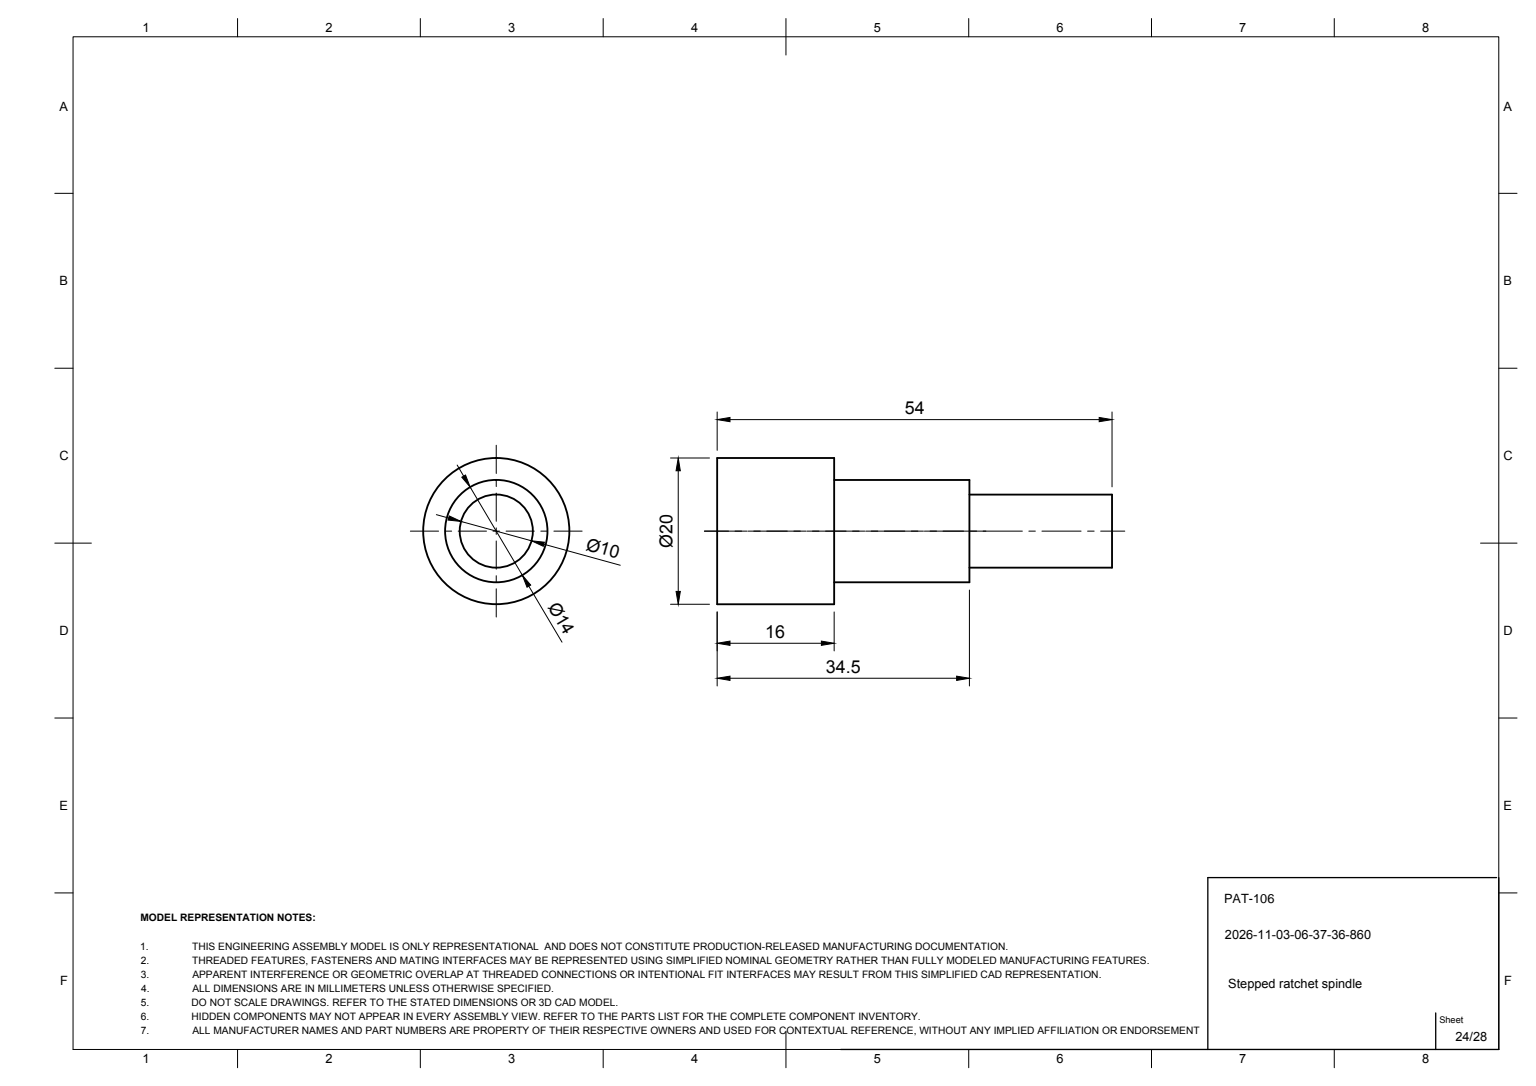
ISO-10303-21;
HEADER;
/* Generated by software containing ST-Developer
 * from STEP Tools, Inc. (www.steptools.com) 
 */

FILE_DESCRIPTION(
/* description */ ('Torsion-spring ratchet demonstrator'),
/* implementation_level */ '2;1');

FILE_NAME(
/* name */ 'Stepped ratchet spindle.step',
/* time_stamp */ '2026-10-29T17:29:17-07:00',
/* author */ (''),
/* organization */ (''),
/* preprocessor_version */ 'ST-DEVELOPER v20.2',
/* originating_system */ 'Autodesk Translation Framework v15.17.0.0',
/* authorisation */ '');

FILE_SCHEMA (('AUTOMOTIVE_DESIGN { 1 0 10303 214 3 1 1 }'));
ENDSEC;

DATA;
#10=MECHANICAL_DESIGN_GEOMETRIC_PRESENTATION_REPRESENTATION('',(#308),#11258);
#252=SHAPE_REPRESENTATION_RELATIONSHIP('SRR','None',#11380,#276);
#276=ADVANCED_BREP_SHAPE_REPRESENTATION('',(#338),#11250);
#308=STYLED_ITEM('',(#11577),#338);
#338=MANIFOLD_SOLID_BREP('Body1',#5181);
#420=FACE_BOUND('',#1196,.T.);
#421=FACE_BOUND('',#1199,.T.);
#530=PLANE('',#5896);
#531=PLANE('',#5901);
#532=PLANE('',#5907);
#533=PLANE('',#5908);
#815=FACE_OUTER_BOUND('',#1195,.T.);
#816=FACE_OUTER_BOUND('',#1197,.T.);
#817=FACE_OUTER_BOUND('',#1198,.T.);
#818=FACE_OUTER_BOUND('',#1200,.T.);
#819=FACE_OUTER_BOUND('',#1201,.T.);
#820=FACE_OUTER_BOUND('',#1202,.T.);
#821=FACE_OUTER_BOUND('',#1203,.T.);
#1195=EDGE_LOOP('',(#4212));
#1196=EDGE_LOOP('',(#4213));
#1197=EDGE_LOOP('',(#4214,#4215,#4216,#4217));
#1198=EDGE_LOOP('',(#4218));
#1199=EDGE_LOOP('',(#4219));
#1200=EDGE_LOOP('',(#4220,#4221,#4222,#4223));
#1201=EDGE_LOOP('',(#4224,#4225,#4226,#4227));
#1202=EDGE_LOOP('',(#4228));
#1203=EDGE_LOOP('',(#4229));
#1481=LINE('',#10498,#1864);
#1482=LINE('',#10505,#1865);
#1483=LINE('',#10508,#1866);
#1864=VECTOR('',#7118,1.);
#1865=VECTOR('',#7127,0.7);
#1866=VECTOR('',#7130,0.5);
#2295=CIRCLE('',#5897,1.);
#2296=CIRCLE('',#5898,0.7);
#2297=CIRCLE('',#5900,1.);
#2298=CIRCLE('',#5902,0.7);
#2299=CIRCLE('',#5903,0.5);
#2300=CIRCLE('',#5906,0.5);
#2599=VERTEX_POINT('',#10491);
#2600=VERTEX_POINT('',#10493);
#2601=VERTEX_POINT('',#10496);
#2602=VERTEX_POINT('',#10500);
#2603=VERTEX_POINT('',#10502);
#2604=VERTEX_POINT('',#10507);
#3166=EDGE_CURVE('',#2599,#2599,#2295,.T.);
#3167=EDGE_CURVE('',#2600,#2600,#2296,.T.);
#3168=EDGE_CURVE('',#2601,#2601,#2297,.T.);
#3169=EDGE_CURVE('',#2601,#2599,#1481,.T.);
#3170=EDGE_CURVE('',#2602,#2602,#2298,.T.);
#3171=EDGE_CURVE('',#2603,#2603,#2299,.T.);
#3172=EDGE_CURVE('',#2600,#2602,#1482,.T.);
#3173=EDGE_CURVE('',#2603,#2604,#1483,.T.);
#3174=EDGE_CURVE('',#2604,#2604,#2300,.T.);
#4212=ORIENTED_EDGE('',*,*,#3166,.F.);
#4213=ORIENTED_EDGE('',*,*,#3167,.T.);
#4214=ORIENTED_EDGE('',*,*,#3168,.F.);
#4215=ORIENTED_EDGE('',*,*,#3169,.T.);
#4216=ORIENTED_EDGE('',*,*,#3166,.T.);
#4217=ORIENTED_EDGE('',*,*,#3169,.F.);
#4218=ORIENTED_EDGE('',*,*,#3170,.F.);
#4219=ORIENTED_EDGE('',*,*,#3171,.F.);
#4220=ORIENTED_EDGE('',*,*,#3167,.F.);
#4221=ORIENTED_EDGE('',*,*,#3172,.T.);
#4222=ORIENTED_EDGE('',*,*,#3170,.T.);
#4223=ORIENTED_EDGE('',*,*,#3172,.F.);
#4224=ORIENTED_EDGE('',*,*,#3171,.T.);
#4225=ORIENTED_EDGE('',*,*,#3173,.T.);
#4226=ORIENTED_EDGE('',*,*,#3174,.T.);
#4227=ORIENTED_EDGE('',*,*,#3173,.F.);
#4228=ORIENTED_EDGE('',*,*,#3168,.T.);
#4229=ORIENTED_EDGE('',*,*,#3174,.F.);
#4832=CYLINDRICAL_SURFACE('',#5899,1.);
#4833=CYLINDRICAL_SURFACE('',#5904,0.7);
#4834=CYLINDRICAL_SURFACE('',#5905,0.5);
#5041=ADVANCED_FACE('',(#815,#420),#530,.F.);
#5042=ADVANCED_FACE('',(#816),#4832,.T.);
#5043=ADVANCED_FACE('',(#817,#421),#531,.F.);
#5044=ADVANCED_FACE('',(#818),#4833,.T.);
#5045=ADVANCED_FACE('',(#819),#4834,.T.);
#5046=ADVANCED_FACE('',(#820),#532,.T.);
#5047=ADVANCED_FACE('',(#821),#533,.F.);
#5181=CLOSED_SHELL('',(#5041,#5042,#5043,#5044,#5045,#5046,#5047));
#5895=AXIS2_PLACEMENT_3D('',#10489,#7106,#7107);
#5896=AXIS2_PLACEMENT_3D('',#10490,#7108,#7109);
#5897=AXIS2_PLACEMENT_3D('',#10492,#7110,#7111);
#5898=AXIS2_PLACEMENT_3D('',#10494,#7112,#7113);
#5899=AXIS2_PLACEMENT_3D('',#10495,#7114,#7115);
#5900=AXIS2_PLACEMENT_3D('',#10497,#7116,#7117);
#5901=AXIS2_PLACEMENT_3D('',#10499,#7119,#7120);
#5902=AXIS2_PLACEMENT_3D('',#10501,#7121,#7122);
#5903=AXIS2_PLACEMENT_3D('',#10503,#7123,#7124);
#5904=AXIS2_PLACEMENT_3D('',#10504,#7125,#7126);
#5905=AXIS2_PLACEMENT_3D('',#10506,#7128,#7129);
#5906=AXIS2_PLACEMENT_3D('',#10509,#7131,#7132);
#5907=AXIS2_PLACEMENT_3D('',#10510,#7133,#7134);
#5908=AXIS2_PLACEMENT_3D('',#10511,#7135,#7136);
#7106=DIRECTION('axis',(0.,0.,1.));
#7107=DIRECTION('refdir',(1.,0.,0.));
#7108=DIRECTION('center_axis',(0.,0.,1.));
#7109=DIRECTION('ref_axis',(1.,0.,0.));
#7110=DIRECTION('center_axis',(0.,0.,1.));
#7111=DIRECTION('ref_axis',(1.,0.,0.));
#7112=DIRECTION('center_axis',(0.,0.,1.));
#7113=DIRECTION('ref_axis',(1.,0.,0.));
#7114=DIRECTION('center_axis',(0.,0.,1.));
#7115=DIRECTION('ref_axis',(1.,0.,0.));
#7116=DIRECTION('center_axis',(0.,0.,1.));
#7117=DIRECTION('ref_axis',(1.,0.,0.));
#7118=DIRECTION('',(0.,0.,-1.));
#7119=DIRECTION('center_axis',(0.,0.,1.));
#7120=DIRECTION('ref_axis',(1.,0.,0.));
#7121=DIRECTION('center_axis',(0.,0.,1.));
#7122=DIRECTION('ref_axis',(1.,0.,0.));
#7123=DIRECTION('center_axis',(0.,0.,-1.));
#7124=DIRECTION('ref_axis',(1.,0.,0.));
#7125=DIRECTION('center_axis',(0.,0.,1.));
#7126=DIRECTION('ref_axis',(1.,0.,0.));
#7127=DIRECTION('',(0.,0.,-1.));
#7128=DIRECTION('center_axis',(0.,0.,1.));
#7129=DIRECTION('ref_axis',(1.,0.,0.));
#7130=DIRECTION('',(0.,0.,-1.));
#7131=DIRECTION('center_axis',(0.,0.,1.));
#7132=DIRECTION('ref_axis',(1.,0.,0.));
#7133=DIRECTION('center_axis',(0.,0.,1.));
#7134=DIRECTION('ref_axis',(1.,0.,0.));
#7135=DIRECTION('center_axis',(0.,0.,1.));
#7136=DIRECTION('ref_axis',(1.,0.,0.));
#10489=CARTESIAN_POINT('',(0.,0.,0.));
#10490=CARTESIAN_POINT('Origin',(0.,0.,4.8));
#10491=CARTESIAN_POINT('',(-1.,-1.22464679914735E-16,4.8));
#10492=CARTESIAN_POINT('Origin',(0.,0.,4.8));
#10493=CARTESIAN_POINT('',(-0.7,-8.57252759403147E-17,4.8));
#10494=CARTESIAN_POINT('Origin',(0.,0.,4.8));
#10495=CARTESIAN_POINT('Origin',(0.,0.,4.8));
#10496=CARTESIAN_POINT('',(-1.,-1.22464679914735E-16,6.4));
#10497=CARTESIAN_POINT('Origin',(0.,0.,6.4));
#10498=CARTESIAN_POINT('',(-1.,-1.22464679914735E-16,4.8));
#10499=CARTESIAN_POINT('Origin',(0.,0.,2.95));
#10500=CARTESIAN_POINT('',(-0.7,-8.57252759403147E-17,2.95));
#10501=CARTESIAN_POINT('Origin',(0.,0.,2.95));
#10502=CARTESIAN_POINT('',(-0.5,6.12323399573677E-17,2.95));
#10503=CARTESIAN_POINT('Origin',(0.,0.,2.95));
#10504=CARTESIAN_POINT('Origin',(0.,0.,2.95));
#10505=CARTESIAN_POINT('',(-0.7,-8.57252759403147E-17,2.95));
#10506=CARTESIAN_POINT('Origin',(0.,0.,1.));
#10507=CARTESIAN_POINT('',(-0.5,-6.12323399573677E-17,1.));
#10508=CARTESIAN_POINT('',(-0.5,-6.12323399573677E-17,1.));
#10509=CARTESIAN_POINT('Origin',(0.,0.,1.));
#10510=CARTESIAN_POINT('Origin',(0.,0.,6.4));
#10511=CARTESIAN_POINT('Origin',(0.,0.,1.));
#11220=UNCERTAINTY_MEASURE_WITH_UNIT(LENGTH_MEASURE(0.001),#11259,
'DISTANCE_ACCURACY_VALUE',
'Maximum model space distance between geometric entities at asserted c
onnectivities');
#11228=UNCERTAINTY_MEASURE_WITH_UNIT(LENGTH_MEASURE(0.001),#11259,
'DISTANCE_ACCURACY_VALUE',
'Maximum model space distance between geometric entities at asserted c
onnectivities');
#11250=(
GEOMETRIC_REPRESENTATION_CONTEXT(3)
GLOBAL_UNCERTAINTY_ASSIGNED_CONTEXT((#11220))
GLOBAL_UNIT_ASSIGNED_CONTEXT((#11259,#11261,#11262))
REPRESENTATION_CONTEXT('','3D')
);
#11258=(
GEOMETRIC_REPRESENTATION_CONTEXT(3)
GLOBAL_UNCERTAINTY_ASSIGNED_CONTEXT((#11228))
GLOBAL_UNIT_ASSIGNED_CONTEXT((#11259,#11261,#11262))
REPRESENTATION_CONTEXT('','3D')
);
#11259=(
LENGTH_UNIT()
NAMED_UNIT(*)
SI_UNIT(.CENTI.,.METRE.)
);
#11261=(
NAMED_UNIT(*)
PLANE_ANGLE_UNIT()
SI_UNIT($,.RADIAN.)
);
#11262=(
NAMED_UNIT(*)
SI_UNIT($,.STERADIAN.)
SOLID_ANGLE_UNIT()
);
#11284=SHAPE_DEFINITION_REPRESENTATION(#11341,#11380);
#11341=PRODUCT_DEFINITION_SHAPE('',$,#11410);
#11380=SHAPE_REPRESENTATION('',(#5895),#11250);
#11388=PRODUCT_DEFINITION_CONTEXT('part definition',#11477,'design');
#11410=PRODUCT_DEFINITION('Stepped ratchet spindle',
'Stepped ratchet spindle',#11439,#11388);
#11439=PRODUCT_DEFINITION_FORMATION('',$,#11500);
#11477=APPLICATION_CONTEXT(
'Core Data for Automotive Mechanical Design Process');
#11478=PRODUCT_CONTEXT('part definition',#11477,'mechanical');
#11500=PRODUCT('Stepped ratchet spindle','Stepped ratchet spindle',
'Stepped ratchet spindle',(#11478));
#11571=COLOUR_RGB('Sky Blue',0.24,0.69,0.87);
#11572=FILL_AREA_STYLE_COLOUR('',#11571);
#11573=FILL_AREA_STYLE('',(#11572));
#11574=SURFACE_STYLE_FILL_AREA(#11573);
#11575=SURFACE_SIDE_STYLE('',(#11574));
#11576=SURFACE_STYLE_USAGE(.BOTH.,#11575);
#11577=PRESENTATION_STYLE_ASSIGNMENT((#11576));
ENDSEC;
END-ISO-10303-21;
